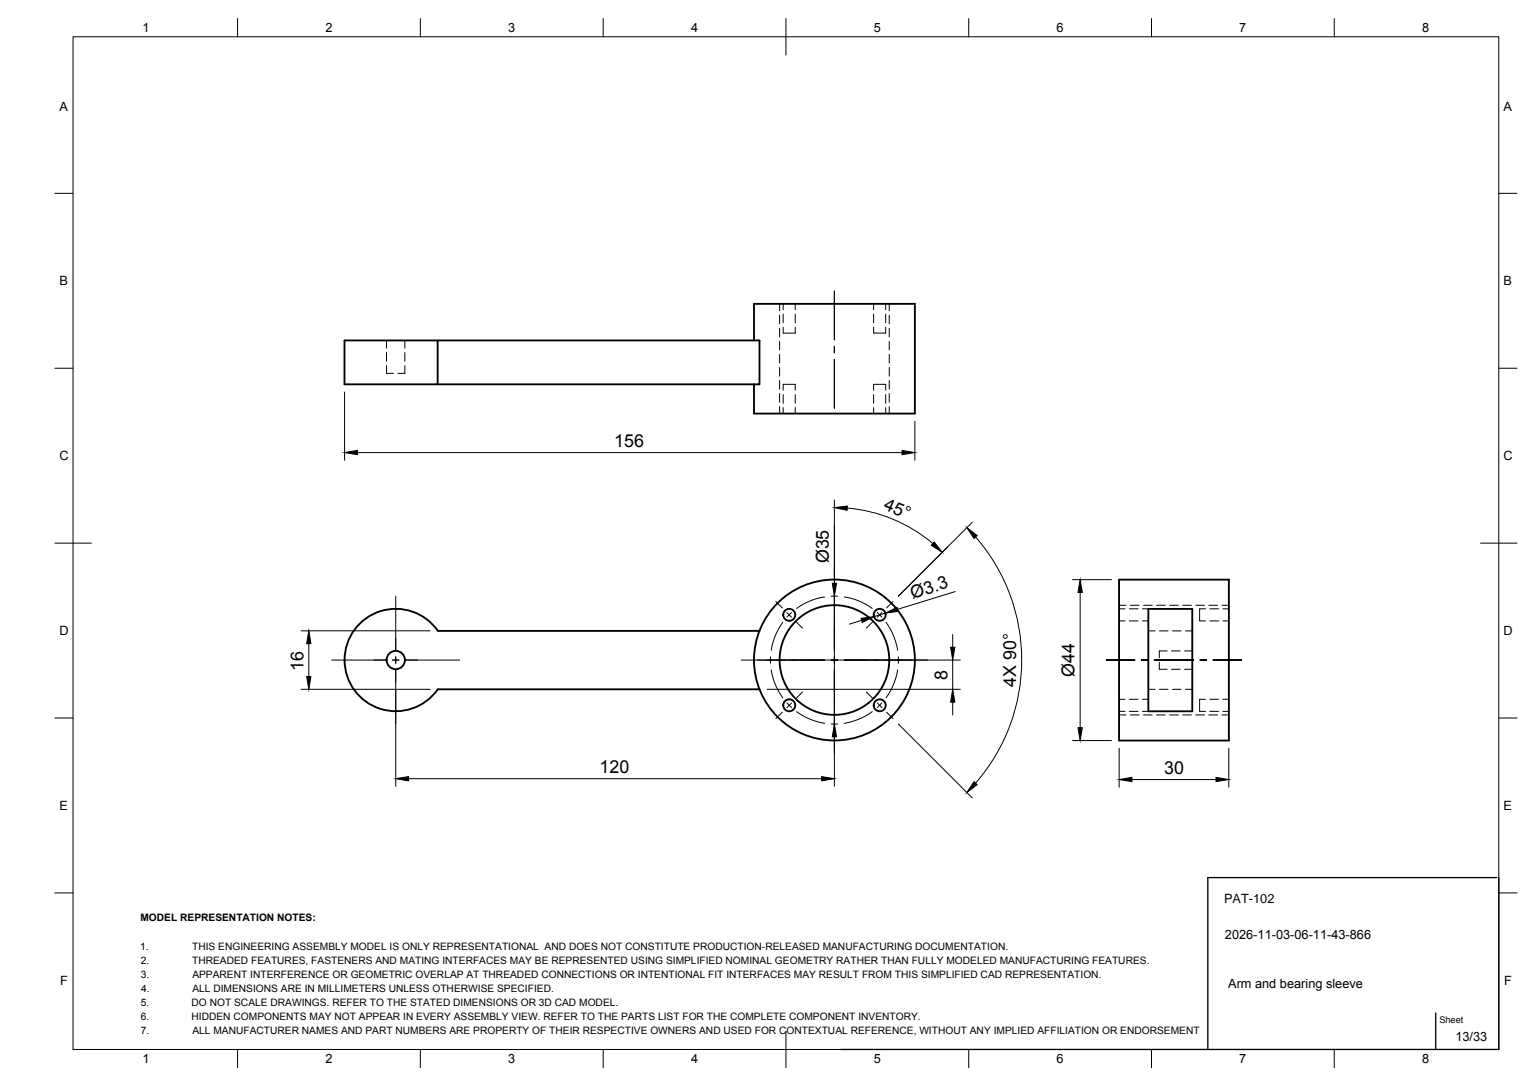
ISO-10303-21;
HEADER;
/* Generated by software containing ST-Developer
 * from STEP Tools, Inc. (www.steptools.com) 
 */

FILE_DESCRIPTION(
/* description */ ('Swing-away clamp arm'),
/* implementation_level */ '2;1');

FILE_NAME(
/* name */ 'Arm and bearing sleeve.step',
/* time_stamp */ '2026-10-28T03:26:03-07:00',
/* author */ (''),
/* organization */ (''),
/* preprocessor_version */ 'ST-DEVELOPER v20.2',
/* originating_system */ 'Autodesk Translation Framework v15.17.0.0',
/* authorisation */ '');

FILE_SCHEMA (('AUTOMOTIVE_DESIGN { 1 0 10303 214 3 1 1 }'));
ENDSEC;

DATA;
#10=MECHANICAL_DESIGN_GEOMETRIC_PRESENTATION_REPRESENTATION('',(#300),#10627);
#248=SHAPE_REPRESENTATION_RELATIONSHIP('SRR','None',#10747,#274);
#274=ADVANCED_BREP_SHAPE_REPRESENTATION('',(#333),#10606);
#300=STYLED_ITEM('',(#10965),#333);
#333=MANIFOLD_SOLID_BREP('Body1',#4907);
#385=FACE_BOUND('',#1095,.T.);
#386=FACE_BOUND('',#1101,.T.);
#387=FACE_BOUND('',#1103,.T.);
#388=FACE_BOUND('',#1104,.T.);
#389=FACE_BOUND('',#1105,.T.);
#390=FACE_BOUND('',#1106,.T.);
#391=FACE_BOUND('',#1107,.T.);
#392=FACE_BOUND('',#1109,.T.);
#393=FACE_BOUND('',#1110,.T.);
#394=FACE_BOUND('',#1111,.T.);
#395=FACE_BOUND('',#1112,.T.);
#396=FACE_BOUND('',#1113,.T.);
#537=PLANE('',#5410);
#538=PLANE('',#5414);
#539=PLANE('',#5418);
#540=PLANE('',#5422);
#541=PLANE('',#5426);
#542=PLANE('',#5430);
#543=PLANE('',#5434);
#544=PLANE('',#5438);
#545=PLANE('',#5442);
#546=PLANE('',#5446);
#547=PLANE('',#5448);
#548=PLANE('',#5449);
#549=PLANE('',#5450);
#550=PLANE('',#5458);
#551=PLANE('',#5459);
#741=FACE_OUTER_BOUND('',#1075,.T.);
#742=FACE_OUTER_BOUND('',#1076,.T.);
#743=FACE_OUTER_BOUND('',#1077,.T.);
#744=FACE_OUTER_BOUND('',#1078,.T.);
#745=FACE_OUTER_BOUND('',#1079,.T.);
#746=FACE_OUTER_BOUND('',#1080,.T.);
#747=FACE_OUTER_BOUND('',#1081,.T.);
#748=FACE_OUTER_BOUND('',#1082,.T.);
#749=FACE_OUTER_BOUND('',#1083,.T.);
#750=FACE_OUTER_BOUND('',#1084,.T.);
#751=FACE_OUTER_BOUND('',#1085,.T.);
#752=FACE_OUTER_BOUND('',#1086,.T.);
#753=FACE_OUTER_BOUND('',#1087,.T.);
#754=FACE_OUTER_BOUND('',#1088,.T.);
#755=FACE_OUTER_BOUND('',#1089,.T.);
#756=FACE_OUTER_BOUND('',#1090,.T.);
#757=FACE_OUTER_BOUND('',#1091,.T.);
#758=FACE_OUTER_BOUND('',#1092,.T.);
#759=FACE_OUTER_BOUND('',#1093,.T.);
#760=FACE_OUTER_BOUND('',#1094,.T.);
#761=FACE_OUTER_BOUND('',#1096,.T.);
#762=FACE_OUTER_BOUND('',#1097,.T.);
#763=FACE_OUTER_BOUND('',#1098,.T.);
#764=FACE_OUTER_BOUND('',#1099,.T.);
#765=FACE_OUTER_BOUND('',#1100,.T.);
#766=FACE_OUTER_BOUND('',#1102,.T.);
#767=FACE_OUTER_BOUND('',#1108,.T.);
#1075=EDGE_LOOP('',(#3759,#3760,#3761,#3762));
#1076=EDGE_LOOP('',(#3763));
#1077=EDGE_LOOP('',(#3764,#3765,#3766,#3767));
#1078=EDGE_LOOP('',(#3768));
#1079=EDGE_LOOP('',(#3769,#3770,#3771,#3772));
#1080=EDGE_LOOP('',(#3773));
#1081=EDGE_LOOP('',(#3774,#3775,#3776,#3777));
#1082=EDGE_LOOP('',(#3778));
#1083=EDGE_LOOP('',(#3779,#3780,#3781,#3782));
#1084=EDGE_LOOP('',(#3783));
#1085=EDGE_LOOP('',(#3784,#3785,#3786,#3787));
#1086=EDGE_LOOP('',(#3788));
#1087=EDGE_LOOP('',(#3789,#3790,#3791,#3792));
#1088=EDGE_LOOP('',(#3793));
#1089=EDGE_LOOP('',(#3794,#3795,#3796,#3797));
#1090=EDGE_LOOP('',(#3798));
#1091=EDGE_LOOP('',(#3799,#3800,#3801,#3802));
#1092=EDGE_LOOP('',(#3803));
#1093=EDGE_LOOP('',(#3804,#3805,#3806,#3807));
#1094=EDGE_LOOP('',(#3808,#3809,#3810,#3811));
#1095=EDGE_LOOP('',(#3812));
#1096=EDGE_LOOP('',(#3813,#3814,#3815,#3816));
#1097=EDGE_LOOP('',(#3817,#3818,#3819,#3820));
#1098=EDGE_LOOP('',(#3821,#3822,#3823,#3824));
#1099=EDGE_LOOP('',(#3825,#3826,#3827,#3828));
#1100=EDGE_LOOP('',(#3829,#3830,#3831,#3832));
#1101=EDGE_LOOP('',(#3833,#3834,#3835,#3836));
#1102=EDGE_LOOP('',(#3837));
#1103=EDGE_LOOP('',(#3838));
#1104=EDGE_LOOP('',(#3839));
#1105=EDGE_LOOP('',(#3840));
#1106=EDGE_LOOP('',(#3841));
#1107=EDGE_LOOP('',(#3842));
#1108=EDGE_LOOP('',(#3843));
#1109=EDGE_LOOP('',(#3844));
#1110=EDGE_LOOP('',(#3845));
#1111=EDGE_LOOP('',(#3846));
#1112=EDGE_LOOP('',(#3847));
#1113=EDGE_LOOP('',(#3848));
#1529=LINE('',#9352,#1851);
#1530=LINE('',#9359,#1852);
#1531=LINE('',#9366,#1853);
#1532=LINE('',#9373,#1854);
#1533=LINE('',#9380,#1855);
#1534=LINE('',#9387,#1856);
#1535=LINE('',#9394,#1857);
#1536=LINE('',#9401,#1858);
#1537=LINE('',#9408,#1859);
#1538=LINE('',#9414,#1860);
#1539=LINE('',#9418,#1861);
#1540=LINE('',#9422,#1862);
#1541=LINE('',#9425,#1863);
#1542=LINE('',#9428,#1864);
#1543=LINE('',#9429,#1865);
#1544=LINE('',#9432,#1866);
#1545=LINE('',#9433,#1867);
#1546=LINE('',#9440,#1868);
#1547=LINE('',#9446,#1869);
#1851=VECTOR('',#6420,0.165);
#1852=VECTOR('',#6429,0.165);
#1853=VECTOR('',#6438,0.165);
#1854=VECTOR('',#6447,0.165);
#1855=VECTOR('',#6456,0.165);
#1856=VECTOR('',#6465,0.165);
#1857=VECTOR('',#6474,0.165);
#1858=VECTOR('',#6483,0.165);
#1859=VECTOR('',#6492,0.25);
#1860=VECTOR('',#6499,1.);
#1861=VECTOR('',#6502,1.);
#1862=VECTOR('',#6507,1.);
#1863=VECTOR('',#6510,1.);
#1864=VECTOR('',#6513,1.);
#1865=VECTOR('',#6514,1.);
#1866=VECTOR('',#6517,1.);
#1867=VECTOR('',#6518,1.);
#1868=VECTOR('',#6527,1.5);
#1869=VECTOR('',#6534,2.2);
#2055=CIRCLE('',#5408,0.165);
#2056=CIRCLE('',#5409,0.165);
#2057=CIRCLE('',#5412,0.165);
#2058=CIRCLE('',#5413,0.165);
#2059=CIRCLE('',#5416,0.165);
#2060=CIRCLE('',#5417,0.165);
#2061=CIRCLE('',#5420,0.165);
#2062=CIRCLE('',#5421,0.165);
#2063=CIRCLE('',#5424,0.165);
#2064=CIRCLE('',#5425,0.165);
#2065=CIRCLE('',#5428,0.165);
#2066=CIRCLE('',#5429,0.165);
#2067=CIRCLE('',#5432,0.165);
#2068=CIRCLE('',#5433,0.165);
#2069=CIRCLE('',#5436,0.165);
#2070=CIRCLE('',#5437,0.165);
#2071=CIRCLE('',#5440,0.25);
#2072=CIRCLE('',#5441,0.25);
#2073=CIRCLE('',#5444,1.4);
#2074=CIRCLE('',#5445,1.4);
#2075=CIRCLE('',#5447,2.2);
#2076=CIRCLE('',#5451,2.2);
#2077=CIRCLE('',#5453,1.5);
#2078=CIRCLE('',#5454,1.5);
#2079=CIRCLE('',#5456,2.2);
#2080=CIRCLE('',#5457,2.2);
#2420=VERTEX_POINT('',#9349);
#2421=VERTEX_POINT('',#9351);
#2422=VERTEX_POINT('',#9356);
#2423=VERTEX_POINT('',#9358);
#2424=VERTEX_POINT('',#9363);
#2425=VERTEX_POINT('',#9365);
#2426=VERTEX_POINT('',#9370);
#2427=VERTEX_POINT('',#9372);
#2428=VERTEX_POINT('',#9377);
#2429=VERTEX_POINT('',#9379);
#2430=VERTEX_POINT('',#9384);
#2431=VERTEX_POINT('',#9386);
#2432=VERTEX_POINT('',#9391);
#2433=VERTEX_POINT('',#9393);
#2434=VERTEX_POINT('',#9398);
#2435=VERTEX_POINT('',#9400);
#2436=VERTEX_POINT('',#9405);
#2437=VERTEX_POINT('',#9407);
#2438=VERTEX_POINT('',#9412);
#2439=VERTEX_POINT('',#9413);
#2440=VERTEX_POINT('',#9415);
#2441=VERTEX_POINT('',#9417);
#2442=VERTEX_POINT('',#9421);
#2443=VERTEX_POINT('',#9423);
#2444=VERTEX_POINT('',#9427);
#2445=VERTEX_POINT('',#9431);
#2446=VERTEX_POINT('',#9437);
#2447=VERTEX_POINT('',#9439);
#2448=VERTEX_POINT('',#9443);
#2449=VERTEX_POINT('',#9445);
#2912=EDGE_CURVE('',#2420,#2420,#2055,.T.);
#2913=EDGE_CURVE('',#2420,#2421,#1529,.T.);
#2914=EDGE_CURVE('',#2421,#2421,#2056,.T.);
#2915=EDGE_CURVE('',#2422,#2422,#2057,.T.);
#2916=EDGE_CURVE('',#2422,#2423,#1530,.T.);
#2917=EDGE_CURVE('',#2423,#2423,#2058,.T.);
#2918=EDGE_CURVE('',#2424,#2424,#2059,.T.);
#2919=EDGE_CURVE('',#2424,#2425,#1531,.T.);
#2920=EDGE_CURVE('',#2425,#2425,#2060,.T.);
#2921=EDGE_CURVE('',#2426,#2426,#2061,.T.);
#2922=EDGE_CURVE('',#2426,#2427,#1532,.T.);
#2923=EDGE_CURVE('',#2427,#2427,#2062,.T.);
#2924=EDGE_CURVE('',#2428,#2428,#2063,.T.);
#2925=EDGE_CURVE('',#2428,#2429,#1533,.T.);
#2926=EDGE_CURVE('',#2429,#2429,#2064,.T.);
#2927=EDGE_CURVE('',#2430,#2430,#2065,.T.);
#2928=EDGE_CURVE('',#2430,#2431,#1534,.T.);
#2929=EDGE_CURVE('',#2431,#2431,#2066,.T.);
#2930=EDGE_CURVE('',#2432,#2432,#2067,.T.);
#2931=EDGE_CURVE('',#2432,#2433,#1535,.T.);
#2932=EDGE_CURVE('',#2433,#2433,#2068,.T.);
#2933=EDGE_CURVE('',#2434,#2434,#2069,.T.);
#2934=EDGE_CURVE('',#2434,#2435,#1536,.T.);
#2935=EDGE_CURVE('',#2435,#2435,#2070,.T.);
#2936=EDGE_CURVE('',#2436,#2436,#2071,.T.);
#2937=EDGE_CURVE('',#2436,#2437,#1537,.T.);
#2938=EDGE_CURVE('',#2437,#2437,#2072,.T.);
#2939=EDGE_CURVE('',#2438,#2439,#1538,.T.);
#2940=EDGE_CURVE('',#2440,#2438,#2073,.T.);
#2941=EDGE_CURVE('',#2441,#2440,#1539,.T.);
#2942=EDGE_CURVE('',#2441,#2439,#2074,.T.);
#2943=EDGE_CURVE('',#2442,#2441,#1540,.T.);
#2944=EDGE_CURVE('',#2443,#2442,#2075,.T.);
#2945=EDGE_CURVE('',#2439,#2443,#1541,.T.);
#2946=EDGE_CURVE('',#2444,#2440,#1542,.T.);
#2947=EDGE_CURVE('',#2442,#2444,#1543,.T.);
#2948=EDGE_CURVE('',#2445,#2443,#1544,.T.);
#2949=EDGE_CURVE('',#2438,#2445,#1545,.T.);
#2950=EDGE_CURVE('',#2444,#2445,#2076,.T.);
#2951=EDGE_CURVE('',#2446,#2446,#2077,.T.);
#2952=EDGE_CURVE('',#2446,#2447,#1546,.T.);
#2953=EDGE_CURVE('',#2447,#2447,#2078,.T.);
#2954=EDGE_CURVE('',#2448,#2448,#2079,.T.);
#2955=EDGE_CURVE('',#2448,#2449,#1547,.T.);
#2956=EDGE_CURVE('',#2449,#2449,#2080,.T.);
#3759=ORIENTED_EDGE('',*,*,#2912,.F.);
#3760=ORIENTED_EDGE('',*,*,#2913,.T.);
#3761=ORIENTED_EDGE('',*,*,#2914,.F.);
#3762=ORIENTED_EDGE('',*,*,#2913,.F.);
#3763=ORIENTED_EDGE('',*,*,#2912,.T.);
#3764=ORIENTED_EDGE('',*,*,#2915,.F.);
#3765=ORIENTED_EDGE('',*,*,#2916,.T.);
#3766=ORIENTED_EDGE('',*,*,#2917,.F.);
#3767=ORIENTED_EDGE('',*,*,#2916,.F.);
#3768=ORIENTED_EDGE('',*,*,#2915,.T.);
#3769=ORIENTED_EDGE('',*,*,#2918,.F.);
#3770=ORIENTED_EDGE('',*,*,#2919,.T.);
#3771=ORIENTED_EDGE('',*,*,#2920,.F.);
#3772=ORIENTED_EDGE('',*,*,#2919,.F.);
#3773=ORIENTED_EDGE('',*,*,#2918,.T.);
#3774=ORIENTED_EDGE('',*,*,#2921,.F.);
#3775=ORIENTED_EDGE('',*,*,#2922,.T.);
#3776=ORIENTED_EDGE('',*,*,#2923,.F.);
#3777=ORIENTED_EDGE('',*,*,#2922,.F.);
#3778=ORIENTED_EDGE('',*,*,#2921,.T.);
#3779=ORIENTED_EDGE('',*,*,#2924,.F.);
#3780=ORIENTED_EDGE('',*,*,#2925,.T.);
#3781=ORIENTED_EDGE('',*,*,#2926,.T.);
#3782=ORIENTED_EDGE('',*,*,#2925,.F.);
#3783=ORIENTED_EDGE('',*,*,#2926,.F.);
#3784=ORIENTED_EDGE('',*,*,#2927,.F.);
#3785=ORIENTED_EDGE('',*,*,#2928,.T.);
#3786=ORIENTED_EDGE('',*,*,#2929,.T.);
#3787=ORIENTED_EDGE('',*,*,#2928,.F.);
#3788=ORIENTED_EDGE('',*,*,#2929,.F.);
#3789=ORIENTED_EDGE('',*,*,#2930,.F.);
#3790=ORIENTED_EDGE('',*,*,#2931,.T.);
#3791=ORIENTED_EDGE('',*,*,#2932,.T.);
#3792=ORIENTED_EDGE('',*,*,#2931,.F.);
#3793=ORIENTED_EDGE('',*,*,#2932,.F.);
#3794=ORIENTED_EDGE('',*,*,#2933,.F.);
#3795=ORIENTED_EDGE('',*,*,#2934,.T.);
#3796=ORIENTED_EDGE('',*,*,#2935,.T.);
#3797=ORIENTED_EDGE('',*,*,#2934,.F.);
#3798=ORIENTED_EDGE('',*,*,#2935,.F.);
#3799=ORIENTED_EDGE('',*,*,#2936,.F.);
#3800=ORIENTED_EDGE('',*,*,#2937,.T.);
#3801=ORIENTED_EDGE('',*,*,#2938,.T.);
#3802=ORIENTED_EDGE('',*,*,#2937,.F.);
#3803=ORIENTED_EDGE('',*,*,#2938,.F.);
#3804=ORIENTED_EDGE('',*,*,#2939,.F.);
#3805=ORIENTED_EDGE('',*,*,#2940,.F.);
#3806=ORIENTED_EDGE('',*,*,#2941,.F.);
#3807=ORIENTED_EDGE('',*,*,#2942,.T.);
#3808=ORIENTED_EDGE('',*,*,#2942,.F.);
#3809=ORIENTED_EDGE('',*,*,#2943,.F.);
#3810=ORIENTED_EDGE('',*,*,#2944,.F.);
#3811=ORIENTED_EDGE('',*,*,#2945,.F.);
#3812=ORIENTED_EDGE('',*,*,#2936,.T.);
#3813=ORIENTED_EDGE('',*,*,#2941,.T.);
#3814=ORIENTED_EDGE('',*,*,#2946,.F.);
#3815=ORIENTED_EDGE('',*,*,#2947,.F.);
#3816=ORIENTED_EDGE('',*,*,#2943,.T.);
#3817=ORIENTED_EDGE('',*,*,#2939,.T.);
#3818=ORIENTED_EDGE('',*,*,#2945,.T.);
#3819=ORIENTED_EDGE('',*,*,#2948,.F.);
#3820=ORIENTED_EDGE('',*,*,#2949,.F.);
#3821=ORIENTED_EDGE('',*,*,#2949,.T.);
#3822=ORIENTED_EDGE('',*,*,#2950,.F.);
#3823=ORIENTED_EDGE('',*,*,#2946,.T.);
#3824=ORIENTED_EDGE('',*,*,#2940,.T.);
#3825=ORIENTED_EDGE('',*,*,#2951,.F.);
#3826=ORIENTED_EDGE('',*,*,#2952,.T.);
#3827=ORIENTED_EDGE('',*,*,#2953,.T.);
#3828=ORIENTED_EDGE('',*,*,#2952,.F.);
#3829=ORIENTED_EDGE('',*,*,#2954,.F.);
#3830=ORIENTED_EDGE('',*,*,#2955,.T.);
#3831=ORIENTED_EDGE('',*,*,#2956,.T.);
#3832=ORIENTED_EDGE('',*,*,#2955,.F.);
#3833=ORIENTED_EDGE('',*,*,#2947,.T.);
#3834=ORIENTED_EDGE('',*,*,#2950,.T.);
#3835=ORIENTED_EDGE('',*,*,#2948,.T.);
#3836=ORIENTED_EDGE('',*,*,#2944,.T.);
#3837=ORIENTED_EDGE('',*,*,#2954,.T.);
#3838=ORIENTED_EDGE('',*,*,#2951,.T.);
#3839=ORIENTED_EDGE('',*,*,#2923,.T.);
#3840=ORIENTED_EDGE('',*,*,#2920,.T.);
#3841=ORIENTED_EDGE('',*,*,#2917,.T.);
#3842=ORIENTED_EDGE('',*,*,#2914,.T.);
#3843=ORIENTED_EDGE('',*,*,#2956,.F.);
#3844=ORIENTED_EDGE('',*,*,#2953,.F.);
#3845=ORIENTED_EDGE('',*,*,#2933,.T.);
#3846=ORIENTED_EDGE('',*,*,#2930,.T.);
#3847=ORIENTED_EDGE('',*,*,#2927,.T.);
#3848=ORIENTED_EDGE('',*,*,#2924,.T.);
#4518=CYLINDRICAL_SURFACE('',#5407,0.165);
#4519=CYLINDRICAL_SURFACE('',#5411,0.165);
#4520=CYLINDRICAL_SURFACE('',#5415,0.165);
#4521=CYLINDRICAL_SURFACE('',#5419,0.165);
#4522=CYLINDRICAL_SURFACE('',#5423,0.165);
#4523=CYLINDRICAL_SURFACE('',#5427,0.165);
#4524=CYLINDRICAL_SURFACE('',#5431,0.165);
#4525=CYLINDRICAL_SURFACE('',#5435,0.165);
#4526=CYLINDRICAL_SURFACE('',#5439,0.25);
#4527=CYLINDRICAL_SURFACE('',#5443,1.4);
#4528=CYLINDRICAL_SURFACE('',#5452,1.5);
#4529=CYLINDRICAL_SURFACE('',#5455,2.2);
#4696=ADVANCED_FACE('',(#741),#4518,.F.);
#4697=ADVANCED_FACE('',(#742),#537,.T.);
#4698=ADVANCED_FACE('',(#743),#4519,.F.);
#4699=ADVANCED_FACE('',(#744),#538,.T.);
#4700=ADVANCED_FACE('',(#745),#4520,.F.);
#4701=ADVANCED_FACE('',(#746),#539,.T.);
#4702=ADVANCED_FACE('',(#747),#4521,.F.);
#4703=ADVANCED_FACE('',(#748),#540,.T.);
#4704=ADVANCED_FACE('',(#749),#4522,.F.);
#4705=ADVANCED_FACE('',(#750),#541,.F.);
#4706=ADVANCED_FACE('',(#751),#4523,.F.);
#4707=ADVANCED_FACE('',(#752),#542,.F.);
#4708=ADVANCED_FACE('',(#753),#4524,.F.);
#4709=ADVANCED_FACE('',(#754),#543,.F.);
#4710=ADVANCED_FACE('',(#755),#4525,.F.);
#4711=ADVANCED_FACE('',(#756),#544,.F.);
#4712=ADVANCED_FACE('',(#757),#4526,.F.);
#4713=ADVANCED_FACE('',(#758),#545,.F.);
#4714=ADVANCED_FACE('',(#759),#4527,.T.);
#4715=ADVANCED_FACE('',(#760,#385),#546,.F.);
#4716=ADVANCED_FACE('',(#761),#547,.T.);
#4717=ADVANCED_FACE('',(#762),#548,.T.);
#4718=ADVANCED_FACE('',(#763),#549,.T.);
#4719=ADVANCED_FACE('',(#764),#4528,.F.);
#4720=ADVANCED_FACE('',(#765,#386),#4529,.T.);
#4721=ADVANCED_FACE('',(#766,#387,#388,#389,#390,#391),#550,.T.);
#4722=ADVANCED_FACE('',(#767,#392,#393,#394,#395,#396),#551,.F.);
#4907=CLOSED_SHELL('',(#4696,#4697,#4698,#4699,#4700,#4701,#4702,#4703,
#4704,#4705,#4706,#4707,#4708,#4709,#4710,#4711,#4712,#4713,#4714,#4715,
#4716,#4717,#4718,#4719,#4720,#4721,#4722));
#5406=AXIS2_PLACEMENT_3D('',#9347,#6414,#6415);
#5407=AXIS2_PLACEMENT_3D('',#9348,#6416,#6417);
#5408=AXIS2_PLACEMENT_3D('',#9350,#6418,#6419);
#5409=AXIS2_PLACEMENT_3D('',#9353,#6421,#6422);
#5410=AXIS2_PLACEMENT_3D('',#9354,#6423,#6424);
#5411=AXIS2_PLACEMENT_3D('',#9355,#6425,#6426);
#5412=AXIS2_PLACEMENT_3D('',#9357,#6427,#6428);
#5413=AXIS2_PLACEMENT_3D('',#9360,#6430,#6431);
#5414=AXIS2_PLACEMENT_3D('',#9361,#6432,#6433);
#5415=AXIS2_PLACEMENT_3D('',#9362,#6434,#6435);
#5416=AXIS2_PLACEMENT_3D('',#9364,#6436,#6437);
#5417=AXIS2_PLACEMENT_3D('',#9367,#6439,#6440);
#5418=AXIS2_PLACEMENT_3D('',#9368,#6441,#6442);
#5419=AXIS2_PLACEMENT_3D('',#9369,#6443,#6444);
#5420=AXIS2_PLACEMENT_3D('',#9371,#6445,#6446);
#5421=AXIS2_PLACEMENT_3D('',#9374,#6448,#6449);
#5422=AXIS2_PLACEMENT_3D('',#9375,#6450,#6451);
#5423=AXIS2_PLACEMENT_3D('',#9376,#6452,#6453);
#5424=AXIS2_PLACEMENT_3D('',#9378,#6454,#6455);
#5425=AXIS2_PLACEMENT_3D('',#9381,#6457,#6458);
#5426=AXIS2_PLACEMENT_3D('',#9382,#6459,#6460);
#5427=AXIS2_PLACEMENT_3D('',#9383,#6461,#6462);
#5428=AXIS2_PLACEMENT_3D('',#9385,#6463,#6464);
#5429=AXIS2_PLACEMENT_3D('',#9388,#6466,#6467);
#5430=AXIS2_PLACEMENT_3D('',#9389,#6468,#6469);
#5431=AXIS2_PLACEMENT_3D('',#9390,#6470,#6471);
#5432=AXIS2_PLACEMENT_3D('',#9392,#6472,#6473);
#5433=AXIS2_PLACEMENT_3D('',#9395,#6475,#6476);
#5434=AXIS2_PLACEMENT_3D('',#9396,#6477,#6478);
#5435=AXIS2_PLACEMENT_3D('',#9397,#6479,#6480);
#5436=AXIS2_PLACEMENT_3D('',#9399,#6481,#6482);
#5437=AXIS2_PLACEMENT_3D('',#9402,#6484,#6485);
#5438=AXIS2_PLACEMENT_3D('',#9403,#6486,#6487);
#5439=AXIS2_PLACEMENT_3D('',#9404,#6488,#6489);
#5440=AXIS2_PLACEMENT_3D('',#9406,#6490,#6491);
#5441=AXIS2_PLACEMENT_3D('',#9409,#6493,#6494);
#5442=AXIS2_PLACEMENT_3D('',#9410,#6495,#6496);
#5443=AXIS2_PLACEMENT_3D('',#9411,#6497,#6498);
#5444=AXIS2_PLACEMENT_3D('',#9416,#6500,#6501);
#5445=AXIS2_PLACEMENT_3D('',#9419,#6503,#6504);
#5446=AXIS2_PLACEMENT_3D('',#9420,#6505,#6506);
#5447=AXIS2_PLACEMENT_3D('',#9424,#6508,#6509);
#5448=AXIS2_PLACEMENT_3D('',#9426,#6511,#6512);
#5449=AXIS2_PLACEMENT_3D('',#9430,#6515,#6516);
#5450=AXIS2_PLACEMENT_3D('',#9434,#6519,#6520);
#5451=AXIS2_PLACEMENT_3D('',#9435,#6521,#6522);
#5452=AXIS2_PLACEMENT_3D('',#9436,#6523,#6524);
#5453=AXIS2_PLACEMENT_3D('',#9438,#6525,#6526);
#5454=AXIS2_PLACEMENT_3D('',#9441,#6528,#6529);
#5455=AXIS2_PLACEMENT_3D('',#9442,#6530,#6531);
#5456=AXIS2_PLACEMENT_3D('',#9444,#6532,#6533);
#5457=AXIS2_PLACEMENT_3D('',#9447,#6535,#6536);
#5458=AXIS2_PLACEMENT_3D('',#9448,#6537,#6538);
#5459=AXIS2_PLACEMENT_3D('',#9449,#6539,#6540);
#6414=DIRECTION('axis',(0.,0.,1.));
#6415=DIRECTION('refdir',(1.,0.,0.));
#6416=DIRECTION('center_axis',(0.,0.,1.));
#6417=DIRECTION('ref_axis',(1.,0.,0.));
#6418=DIRECTION('center_axis',(0.,0.,1.));
#6419=DIRECTION('ref_axis',(1.,0.,0.));
#6420=DIRECTION('',(0.,0.,1.));
#6421=DIRECTION('center_axis',(0.,0.,-1.));
#6422=DIRECTION('ref_axis',(1.,0.,0.));
#6423=DIRECTION('center_axis',(0.,0.,1.));
#6424=DIRECTION('ref_axis',(1.,0.,0.));
#6425=DIRECTION('center_axis',(0.,0.,1.));
#6426=DIRECTION('ref_axis',(1.,0.,0.));
#6427=DIRECTION('center_axis',(0.,0.,1.));
#6428=DIRECTION('ref_axis',(1.,0.,0.));
#6429=DIRECTION('',(0.,0.,1.));
#6430=DIRECTION('center_axis',(0.,0.,-1.));
#6431=DIRECTION('ref_axis',(1.,0.,0.));
#6432=DIRECTION('center_axis',(0.,0.,1.));
#6433=DIRECTION('ref_axis',(1.,0.,0.));
#6434=DIRECTION('center_axis',(0.,0.,1.));
#6435=DIRECTION('ref_axis',(1.,0.,0.));
#6436=DIRECTION('center_axis',(0.,0.,1.));
#6437=DIRECTION('ref_axis',(1.,0.,0.));
#6438=DIRECTION('',(0.,0.,1.));
#6439=DIRECTION('center_axis',(0.,0.,-1.));
#6440=DIRECTION('ref_axis',(1.,0.,0.));
#6441=DIRECTION('center_axis',(0.,0.,1.));
#6442=DIRECTION('ref_axis',(1.,0.,0.));
#6443=DIRECTION('center_axis',(0.,0.,1.));
#6444=DIRECTION('ref_axis',(1.,0.,0.));
#6445=DIRECTION('center_axis',(0.,0.,1.));
#6446=DIRECTION('ref_axis',(1.,0.,0.));
#6447=DIRECTION('',(0.,0.,1.));
#6448=DIRECTION('center_axis',(0.,0.,-1.));
#6449=DIRECTION('ref_axis',(1.,0.,0.));
#6450=DIRECTION('center_axis',(0.,0.,1.));
#6451=DIRECTION('ref_axis',(1.,0.,0.));
#6452=DIRECTION('center_axis',(0.,0.,1.));
#6453=DIRECTION('ref_axis',(1.,0.,0.));
#6454=DIRECTION('center_axis',(0.,0.,1.));
#6455=DIRECTION('ref_axis',(1.,0.,0.));
#6456=DIRECTION('',(0.,0.,1.));
#6457=DIRECTION('center_axis',(0.,0.,1.));
#6458=DIRECTION('ref_axis',(1.,0.,0.));
#6459=DIRECTION('center_axis',(0.,0.,1.));
#6460=DIRECTION('ref_axis',(1.,0.,0.));
#6461=DIRECTION('center_axis',(0.,0.,1.));
#6462=DIRECTION('ref_axis',(1.,0.,0.));
#6463=DIRECTION('center_axis',(0.,0.,1.));
#6464=DIRECTION('ref_axis',(1.,0.,0.));
#6465=DIRECTION('',(0.,0.,1.));
#6466=DIRECTION('center_axis',(0.,0.,1.));
#6467=DIRECTION('ref_axis',(1.,0.,0.));
#6468=DIRECTION('center_axis',(0.,0.,1.));
#6469=DIRECTION('ref_axis',(1.,0.,0.));
#6470=DIRECTION('center_axis',(0.,0.,1.));
#6471=DIRECTION('ref_axis',(1.,0.,0.));
#6472=DIRECTION('center_axis',(0.,0.,1.));
#6473=DIRECTION('ref_axis',(1.,0.,0.));
#6474=DIRECTION('',(0.,0.,1.));
#6475=DIRECTION('center_axis',(0.,0.,1.));
#6476=DIRECTION('ref_axis',(1.,0.,0.));
#6477=DIRECTION('center_axis',(0.,0.,1.));
#6478=DIRECTION('ref_axis',(1.,0.,0.));
#6479=DIRECTION('center_axis',(0.,0.,1.));
#6480=DIRECTION('ref_axis',(1.,0.,0.));
#6481=DIRECTION('center_axis',(0.,0.,1.));
#6482=DIRECTION('ref_axis',(1.,0.,0.));
#6483=DIRECTION('',(0.,0.,1.));
#6484=DIRECTION('center_axis',(0.,0.,1.));
#6485=DIRECTION('ref_axis',(1.,0.,0.));
#6486=DIRECTION('center_axis',(0.,0.,1.));
#6487=DIRECTION('ref_axis',(1.,0.,0.));
#6488=DIRECTION('center_axis',(0.,0.,1.));
#6489=DIRECTION('ref_axis',(1.,0.,0.));
#6490=DIRECTION('center_axis',(0.,0.,1.));
#6491=DIRECTION('ref_axis',(1.,0.,0.));
#6492=DIRECTION('',(0.,0.,1.));
#6493=DIRECTION('center_axis',(0.,0.,1.));
#6494=DIRECTION('ref_axis',(1.,0.,0.));
#6495=DIRECTION('center_axis',(0.,0.,1.));
#6496=DIRECTION('ref_axis',(1.,0.,0.));
#6497=DIRECTION('center_axis',(0.,0.,1.));
#6498=DIRECTION('ref_axis',(1.,0.,0.));
#6499=DIRECTION('',(0.,0.,-1.));
#6500=DIRECTION('center_axis',(0.,0.,1.));
#6501=DIRECTION('ref_axis',(1.,0.,0.));
#6502=DIRECTION('',(0.,0.,1.));
#6503=DIRECTION('center_axis',(0.,0.,1.));
#6504=DIRECTION('ref_axis',(1.,0.,0.));
#6505=DIRECTION('center_axis',(0.,0.,1.));
#6506=DIRECTION('ref_axis',(1.,0.,0.));
#6507=DIRECTION('',(1.,0.,0.));
#6508=DIRECTION('center_axis',(0.,0.,-1.));
#6509=DIRECTION('ref_axis',(1.,0.,0.));
#6510=DIRECTION('',(-1.,0.,0.));
#6511=DIRECTION('center_axis',(0.,-1.,0.));
#6512=DIRECTION('ref_axis',(1.,0.,0.));
#6513=DIRECTION('',(1.,0.,0.));
#6514=DIRECTION('',(0.,0.,1.));
#6515=DIRECTION('center_axis',(0.,1.,0.));
#6516=DIRECTION('ref_axis',(-1.,0.,0.));
#6517=DIRECTION('',(0.,0.,-1.));
#6518=DIRECTION('',(-1.,0.,0.));
#6519=DIRECTION('center_axis',(0.,0.,1.));
#6520=DIRECTION('ref_axis',(1.,0.,0.));
#6521=DIRECTION('center_axis',(0.,0.,1.));
#6522=DIRECTION('ref_axis',(1.,0.,0.));
#6523=DIRECTION('center_axis',(0.,0.,1.));
#6524=DIRECTION('ref_axis',(1.,0.,0.));
#6525=DIRECTION('center_axis',(0.,0.,-1.));
#6526=DIRECTION('ref_axis',(1.,0.,0.));
#6527=DIRECTION('',(0.,0.,-1.));
#6528=DIRECTION('center_axis',(0.,0.,-1.));
#6529=DIRECTION('ref_axis',(1.,0.,0.));
#6530=DIRECTION('center_axis',(0.,0.,1.));
#6531=DIRECTION('ref_axis',(1.,0.,0.));
#6532=DIRECTION('center_axis',(0.,0.,1.));
#6533=DIRECTION('ref_axis',(1.,0.,0.));
#6534=DIRECTION('',(0.,0.,-1.));
#6535=DIRECTION('center_axis',(0.,0.,1.));
#6536=DIRECTION('ref_axis',(1.,0.,0.));
#6537=DIRECTION('center_axis',(0.,0.,1.));
#6538=DIRECTION('ref_axis',(1.,0.,0.));
#6539=DIRECTION('center_axis',(0.,0.,1.));
#6540=DIRECTION('ref_axis',(1.,0.,0.));
#9347=CARTESIAN_POINT('',(0.,0.,0.));
#9348=CARTESIAN_POINT('Origin',(-1.23743686707646,-1.23743686707646,8.2));
#9349=CARTESIAN_POINT('',(-1.40243686707646,-1.23743686707646,8.2));
#9350=CARTESIAN_POINT('Origin',(-1.23743686707646,-1.23743686707646,8.2));
#9351=CARTESIAN_POINT('',(-1.40243686707646,-1.23743686707646,9.));
#9352=CARTESIAN_POINT('',(-1.40243686707646,-1.23743686707646,8.2));
#9353=CARTESIAN_POINT('Origin',(-1.23743686707646,-1.23743686707646,9.));
#9354=CARTESIAN_POINT('Origin',(-1.23743686707646,-1.23743686707646,8.2));
#9355=CARTESIAN_POINT('Origin',(-1.23743686707646,1.23743686707646,8.2));
#9356=CARTESIAN_POINT('',(-1.40243686707646,1.23743686707646,8.2));
#9357=CARTESIAN_POINT('Origin',(-1.23743686707646,1.23743686707646,8.2));
#9358=CARTESIAN_POINT('',(-1.40243686707646,1.23743686707646,9.));
#9359=CARTESIAN_POINT('',(-1.40243686707646,1.23743686707646,8.2));
#9360=CARTESIAN_POINT('Origin',(-1.23743686707646,1.23743686707646,9.));
#9361=CARTESIAN_POINT('Origin',(-1.23743686707646,1.23743686707646,8.2));
#9362=CARTESIAN_POINT('Origin',(1.23743686707646,1.23743686707646,8.2));
#9363=CARTESIAN_POINT('',(1.07243686707646,1.23743686707646,8.2));
#9364=CARTESIAN_POINT('Origin',(1.23743686707646,1.23743686707646,8.2));
#9365=CARTESIAN_POINT('',(1.07243686707646,1.23743686707646,9.));
#9366=CARTESIAN_POINT('',(1.07243686707646,1.23743686707646,8.2));
#9367=CARTESIAN_POINT('Origin',(1.23743686707646,1.23743686707646,9.));
#9368=CARTESIAN_POINT('Origin',(1.23743686707646,1.23743686707646,8.2));
#9369=CARTESIAN_POINT('Origin',(1.23743686707646,-1.23743686707646,8.2));
#9370=CARTESIAN_POINT('',(1.07243686707646,-1.23743686707646,8.2));
#9371=CARTESIAN_POINT('Origin',(1.23743686707646,-1.23743686707646,8.2));
#9372=CARTESIAN_POINT('',(1.07243686707646,-1.23743686707646,9.));
#9373=CARTESIAN_POINT('',(1.07243686707646,-1.23743686707646,8.2));
#9374=CARTESIAN_POINT('Origin',(1.23743686707646,-1.23743686707646,9.));
#9375=CARTESIAN_POINT('Origin',(1.23743686707646,-1.23743686707646,8.2));
#9376=CARTESIAN_POINT('Origin',(-1.23743686707646,-1.23743686707646,5.9));
#9377=CARTESIAN_POINT('',(-1.40243686707646,-1.23743686707646,6.));
#9378=CARTESIAN_POINT('Origin',(-1.23743686707646,-1.23743686707646,6.));
#9379=CARTESIAN_POINT('',(-1.40243686707646,-1.23743686707646,6.8));
#9380=CARTESIAN_POINT('',(-1.40243686707646,-1.23743686707646,5.9));
#9381=CARTESIAN_POINT('Origin',(-1.23743686707646,-1.23743686707646,6.8));
#9382=CARTESIAN_POINT('Origin',(-1.23743686707646,-1.23743686707646,6.8));
#9383=CARTESIAN_POINT('Origin',(-1.23743686707646,1.23743686707646,5.9));
#9384=CARTESIAN_POINT('',(-1.40243686707646,1.23743686707646,6.));
#9385=CARTESIAN_POINT('Origin',(-1.23743686707646,1.23743686707646,6.));
#9386=CARTESIAN_POINT('',(-1.40243686707646,1.23743686707646,6.8));
#9387=CARTESIAN_POINT('',(-1.40243686707646,1.23743686707646,5.9));
#9388=CARTESIAN_POINT('Origin',(-1.23743686707646,1.23743686707646,6.8));
#9389=CARTESIAN_POINT('Origin',(-1.23743686707646,1.23743686707646,6.8));
#9390=CARTESIAN_POINT('Origin',(1.23743686707646,1.23743686707646,5.9));
#9391=CARTESIAN_POINT('',(1.07243686707646,1.23743686707646,6.));
#9392=CARTESIAN_POINT('Origin',(1.23743686707646,1.23743686707646,6.));
#9393=CARTESIAN_POINT('',(1.07243686707646,1.23743686707646,6.8));
#9394=CARTESIAN_POINT('',(1.07243686707646,1.23743686707646,5.9));
#9395=CARTESIAN_POINT('Origin',(1.23743686707646,1.23743686707646,6.8));
#9396=CARTESIAN_POINT('Origin',(1.23743686707646,1.23743686707646,6.8));
#9397=CARTESIAN_POINT('Origin',(1.23743686707646,-1.23743686707646,5.9));
#9398=CARTESIAN_POINT('',(1.07243686707646,-1.23743686707646,6.));
#9399=CARTESIAN_POINT('Origin',(1.23743686707646,-1.23743686707646,6.));
#9400=CARTESIAN_POINT('',(1.07243686707646,-1.23743686707646,6.8));
#9401=CARTESIAN_POINT('',(1.07243686707646,-1.23743686707646,5.9));
#9402=CARTESIAN_POINT('Origin',(1.23743686707646,-1.23743686707646,6.8));
#9403=CARTESIAN_POINT('Origin',(1.23743686707646,-1.23743686707646,6.8));
#9404=CARTESIAN_POINT('Origin',(12.,0.,6.9));
#9405=CARTESIAN_POINT('',(11.75,-3.06161699786838E-17,7.));
#9406=CARTESIAN_POINT('Origin',(12.,0.,7.));
#9407=CARTESIAN_POINT('',(11.75,-3.06161699786838E-17,7.9));
#9408=CARTESIAN_POINT('',(11.75,-3.06161699786838E-17,6.9));
#9409=CARTESIAN_POINT('Origin',(12.,0.,7.9));
#9410=CARTESIAN_POINT('Origin',(12.,0.,7.9));
#9411=CARTESIAN_POINT('Origin',(12.,0.,7.));
#9412=CARTESIAN_POINT('',(10.8510874706924,0.8,8.2));
#9413=CARTESIAN_POINT('',(10.8510874706924,0.8,7.));
#9414=CARTESIAN_POINT('',(10.8510874706924,0.8,7.));
#9415=CARTESIAN_POINT('',(10.8510874706924,-0.8,8.2));
#9416=CARTESIAN_POINT('Origin',(12.,0.,8.2));
#9417=CARTESIAN_POINT('',(10.8510874706924,-0.8,7.));
#9418=CARTESIAN_POINT('',(10.8510874706924,-0.8,7.));
#9419=CARTESIAN_POINT('Origin',(12.,0.,7.));
#9420=CARTESIAN_POINT('Origin',(6.,0.,7.));
#9421=CARTESIAN_POINT('',(2.04939015319192,-0.8,7.));
#9422=CARTESIAN_POINT('',(0.,-0.8,7.));
#9423=CARTESIAN_POINT('',(2.04939015319192,0.8,7.));
#9424=CARTESIAN_POINT('Origin',(0.,0.,7.));
#9425=CARTESIAN_POINT('',(12.,0.8,7.));
#9426=CARTESIAN_POINT('Origin',(0.,-0.8,7.));
#9427=CARTESIAN_POINT('',(2.04939015319192,-0.8,8.2));
#9428=CARTESIAN_POINT('',(0.,-0.8,8.2));
#9429=CARTESIAN_POINT('',(2.04939015319192,-0.8,6.));
#9430=CARTESIAN_POINT('Origin',(12.,0.8,7.));
#9431=CARTESIAN_POINT('',(2.04939015319192,0.8,8.2));
#9432=CARTESIAN_POINT('',(2.04939015319192,0.8,6.));
#9433=CARTESIAN_POINT('',(12.,0.8,8.2));
#9434=CARTESIAN_POINT('Origin',(6.,0.,8.2));
#9435=CARTESIAN_POINT('Origin',(0.,0.,8.2));
#9436=CARTESIAN_POINT('Origin',(0.,0.,6.));
#9437=CARTESIAN_POINT('',(-1.5,-1.83697019872103E-16,9.));
#9438=CARTESIAN_POINT('Origin',(0.,0.,9.));
#9439=CARTESIAN_POINT('',(-1.5,-1.83697019872103E-16,6.));
#9440=CARTESIAN_POINT('',(-1.5,-1.83697019872103E-16,6.));
#9441=CARTESIAN_POINT('Origin',(0.,0.,6.));
#9442=CARTESIAN_POINT('Origin',(0.,0.,6.));
#9443=CARTESIAN_POINT('',(-2.2,-2.69422295812418E-16,9.));
#9444=CARTESIAN_POINT('Origin',(0.,0.,9.));
#9445=CARTESIAN_POINT('',(-2.2,-2.69422295812418E-16,6.));
#9446=CARTESIAN_POINT('',(-2.2,-2.69422295812418E-16,6.));
#9447=CARTESIAN_POINT('Origin',(0.,0.,6.));
#9448=CARTESIAN_POINT('Origin',(0.,0.,9.));
#9449=CARTESIAN_POINT('Origin',(0.,0.,6.));
#10574=UNCERTAINTY_MEASURE_WITH_UNIT(LENGTH_MEASURE(0.001),#10628,
'DISTANCE_ACCURACY_VALUE',
'Maximum model space distance between geometric entities at asserted c
onnectivities');
#10595=UNCERTAINTY_MEASURE_WITH_UNIT(LENGTH_MEASURE(0.001),#10628,
'DISTANCE_ACCURACY_VALUE',
'Maximum model space distance between geometric entities at asserted c
onnectivities');
#10606=(
GEOMETRIC_REPRESENTATION_CONTEXT(3)
GLOBAL_UNCERTAINTY_ASSIGNED_CONTEXT((#10574))
GLOBAL_UNIT_ASSIGNED_CONTEXT((#10628,#10630,#10631))
REPRESENTATION_CONTEXT('','3D')
);
#10627=(
GEOMETRIC_REPRESENTATION_CONTEXT(3)
GLOBAL_UNCERTAINTY_ASSIGNED_CONTEXT((#10595))
GLOBAL_UNIT_ASSIGNED_CONTEXT((#10628,#10630,#10631))
REPRESENTATION_CONTEXT('','3D')
);
#10628=(
LENGTH_UNIT()
NAMED_UNIT(*)
SI_UNIT(.CENTI.,.METRE.)
);
#10630=(
NAMED_UNIT(*)
PLANE_ANGLE_UNIT()
SI_UNIT($,.RADIAN.)
);
#10631=(
NAMED_UNIT(*)
SI_UNIT($,.STERADIAN.)
SOLID_ANGLE_UNIT()
);
#10642=SHAPE_DEFINITION_REPRESENTATION(#10683,#10747);
#10683=PRODUCT_DEFINITION_SHAPE('',$,#10779);
#10747=SHAPE_REPRESENTATION('',(#5406),#10606);
#10768=PRODUCT_DEFINITION_CONTEXT('part definition',#10863,'design');
#10779=PRODUCT_DEFINITION('Arm and bearing sleeve',
'Arm and bearing sleeve',#10810,#10768);
#10810=PRODUCT_DEFINITION_FORMATION('',$,#10875);
#10863=APPLICATION_CONTEXT(
'Core Data for Automotive Mechanical Design Process');
#10864=PRODUCT_CONTEXT('part definition',#10863,'mechanical');
#10875=PRODUCT('Arm and bearing sleeve','Arm and bearing sleeve',
'Arm and bearing sleeve',(#10864));
#10959=COLOUR_RGB('Grey',0.48,0.52,0.57);
#10960=FILL_AREA_STYLE_COLOUR('',#10959);
#10961=FILL_AREA_STYLE('',(#10960));
#10962=SURFACE_STYLE_FILL_AREA(#10961);
#10963=SURFACE_SIDE_STYLE('',(#10962));
#10964=SURFACE_STYLE_USAGE(.BOTH.,#10963);
#10965=PRESENTATION_STYLE_ASSIGNMENT((#10964));
ENDSEC;
END-ISO-10303-21;
